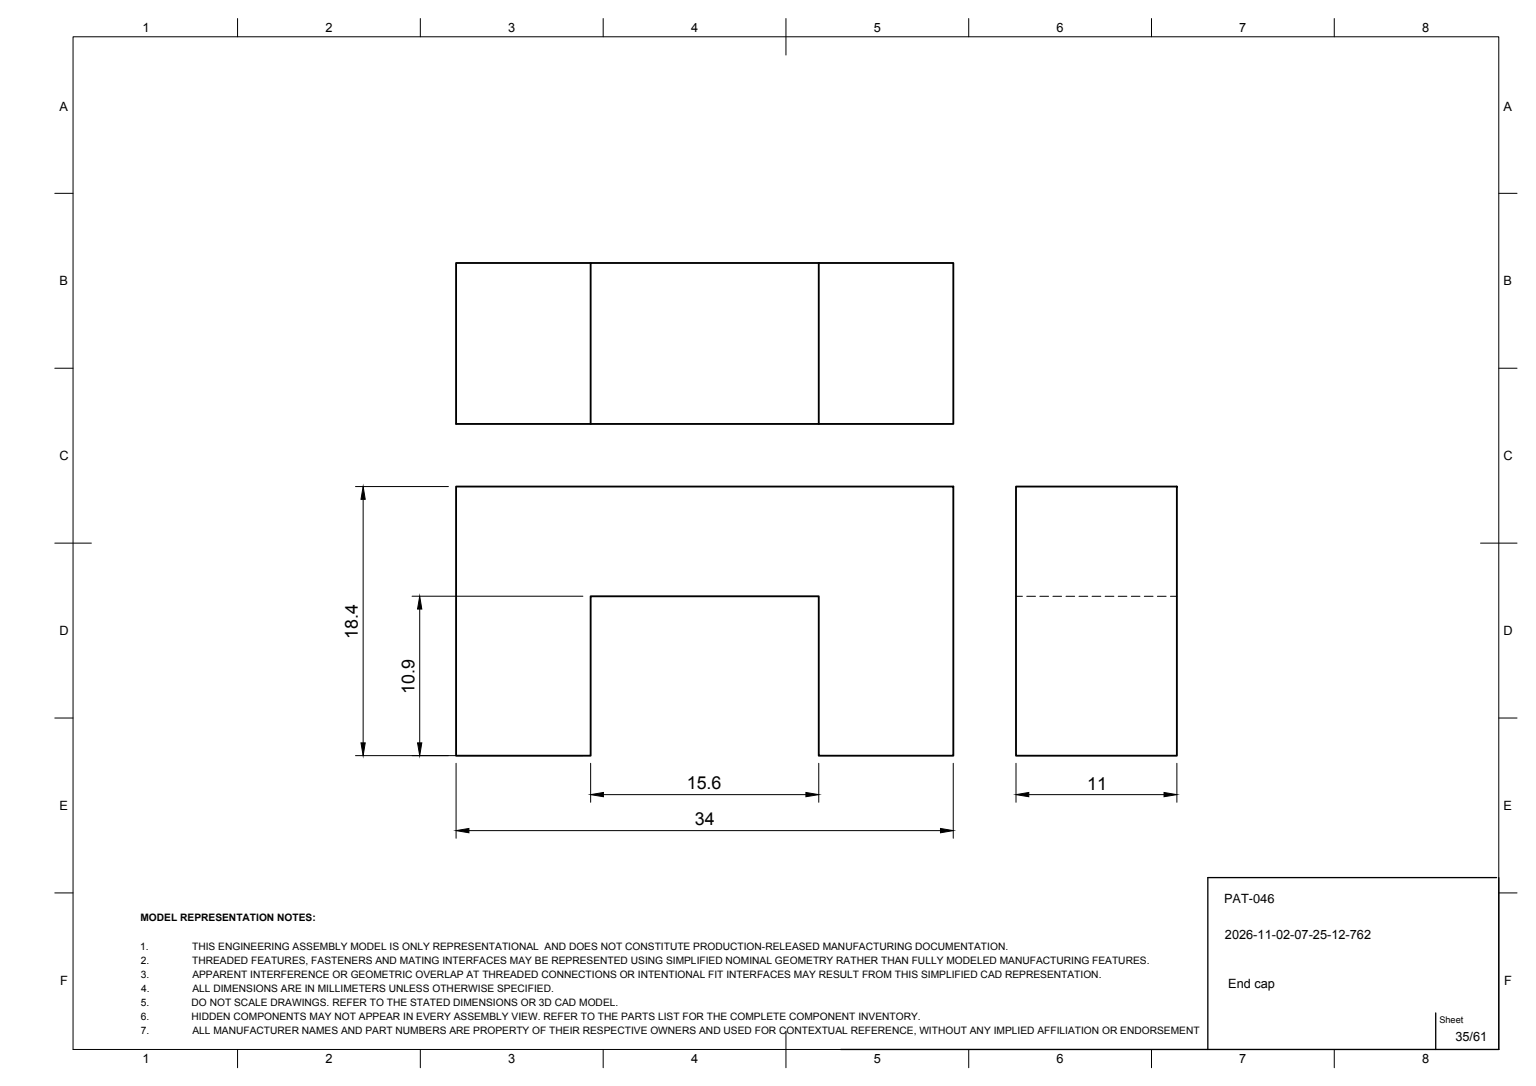
ISO-10303-21;
HEADER;
/* Generated by software containing ST-Developer
 * from STEP Tools, Inc. (www.steptools.com) 
 */

FILE_DESCRIPTION(
/* description */ ('Gear mesh backlash fixture'),
/* implementation_level */ '2;1');

FILE_NAME(
/* name */ 'End cap.step',
/* time_stamp */ '2026-10-28T03:26:00-07:00',
/* author */ (''),
/* organization */ (''),
/* preprocessor_version */ 'ST-DEVELOPER v20.2',
/* originating_system */ 'Autodesk Translation Framework v15.17.0.0',
/* authorisation */ '');

FILE_SCHEMA (('AUTOMOTIVE_DESIGN { 1 0 10303 214 3 1 1 }'));
ENDSEC;

DATA;
#10=MECHANICAL_DESIGN_GEOMETRIC_PRESENTATION_REPRESENTATION('',(#1048),#57900);
#941=SHAPE_REPRESENTATION_RELATIONSHIP('SRR','None',#58139,#991);
#991=ADVANCED_BREP_SHAPE_REPRESENTATION('',(#1112),#57872);
#1048=STYLED_ITEM('',(#58479),#1112);
#1112=MANIFOLD_SOLID_BREP('Body1',#13609);
#1502=PLANE('',#14853);
#1503=PLANE('',#14854);
#1504=PLANE('',#14855);
#1505=PLANE('',#14856);
#1506=PLANE('',#14857);
#1507=PLANE('',#14858);
#1508=PLANE('',#14859);
#1509=PLANE('',#14860);
#1510=PLANE('',#14861);
#1511=PLANE('',#14862);
#2006=FACE_OUTER_BOUND('',#2908,.T.);
#2007=FACE_OUTER_BOUND('',#2909,.T.);
#2008=FACE_OUTER_BOUND('',#2910,.T.);
#2009=FACE_OUTER_BOUND('',#2911,.T.);
#2010=FACE_OUTER_BOUND('',#2912,.T.);
#2011=FACE_OUTER_BOUND('',#2913,.T.);
#2012=FACE_OUTER_BOUND('',#2914,.T.);
#2013=FACE_OUTER_BOUND('',#2915,.T.);
#2014=FACE_OUTER_BOUND('',#2916,.T.);
#2015=FACE_OUTER_BOUND('',#2917,.T.);
#2908=EDGE_LOOP('',(#10317,#10318,#10319,#10320));
#2909=EDGE_LOOP('',(#10321,#10322,#10323,#10324));
#2910=EDGE_LOOP('',(#10325,#10326,#10327,#10328));
#2911=EDGE_LOOP('',(#10329,#10330,#10331,#10332));
#2912=EDGE_LOOP('',(#10333,#10334,#10335,#10336));
#2913=EDGE_LOOP('',(#10337,#10338,#10339,#10340));
#2914=EDGE_LOOP('',(#10341,#10342,#10343,#10344));
#2915=EDGE_LOOP('',(#10345,#10346,#10347,#10348));
#2916=EDGE_LOOP('',(#10349,#10350,#10351,#10352,#10353,#10354,#10355,#10356));
#2917=EDGE_LOOP('',(#10357,#10358,#10359,#10360,#10361,#10362,#10363,#10364));
#3795=LINE('',#21242,#4684);
#3796=LINE('',#21244,#4685);
#3797=LINE('',#21246,#4686);
#3798=LINE('',#21247,#4687);
#3799=LINE('',#21250,#4688);
#3800=LINE('',#21252,#4689);
#3801=LINE('',#21253,#4690);
#3802=LINE('',#21256,#4691);
#3803=LINE('',#21258,#4692);
#3804=LINE('',#21259,#4693);
#3805=LINE('',#21262,#4694);
#3806=LINE('',#21264,#4695);
#3807=LINE('',#21265,#4696);
#3808=LINE('',#21268,#4697);
#3809=LINE('',#21270,#4698);
#3810=LINE('',#21271,#4699);
#3811=LINE('',#21274,#4700);
#3812=LINE('',#21276,#4701);
#3813=LINE('',#21277,#4702);
#3814=LINE('',#21280,#4703);
#3815=LINE('',#21282,#4704);
#3816=LINE('',#21283,#4705);
#3817=LINE('',#21285,#4706);
#3818=LINE('',#21286,#4707);
#4684=VECTOR('',#17280,1.);
#4685=VECTOR('',#17281,1.);
#4686=VECTOR('',#17282,1.);
#4687=VECTOR('',#17283,1.);
#4688=VECTOR('',#17286,1.);
#4689=VECTOR('',#17287,1.);
#4690=VECTOR('',#17288,1.);
#4691=VECTOR('',#17291,1.);
#4692=VECTOR('',#17292,1.);
#4693=VECTOR('',#17293,1.);
#4694=VECTOR('',#17296,1.);
#4695=VECTOR('',#17297,1.);
#4696=VECTOR('',#17298,1.);
#4697=VECTOR('',#17301,1.);
#4698=VECTOR('',#17302,1.);
#4699=VECTOR('',#17303,1.);
#4700=VECTOR('',#17306,1.);
#4701=VECTOR('',#17307,1.);
#4702=VECTOR('',#17308,1.);
#4703=VECTOR('',#17311,1.);
#4704=VECTOR('',#17312,1.);
#4705=VECTOR('',#17313,1.);
#4706=VECTOR('',#17316,1.);
#4707=VECTOR('',#17317,1.);
#6263=VERTEX_POINT('',#21240);
#6264=VERTEX_POINT('',#21241);
#6265=VERTEX_POINT('',#21243);
#6266=VERTEX_POINT('',#21245);
#6267=VERTEX_POINT('',#21249);
#6268=VERTEX_POINT('',#21251);
#6269=VERTEX_POINT('',#21255);
#6270=VERTEX_POINT('',#21257);
#6271=VERTEX_POINT('',#21261);
#6272=VERTEX_POINT('',#21263);
#6273=VERTEX_POINT('',#21267);
#6274=VERTEX_POINT('',#21269);
#6275=VERTEX_POINT('',#21273);
#6276=VERTEX_POINT('',#21275);
#6277=VERTEX_POINT('',#21279);
#6278=VERTEX_POINT('',#21281);
#7745=EDGE_CURVE('',#6263,#6264,#3795,.T.);
#7746=EDGE_CURVE('',#6263,#6265,#3796,.T.);
#7747=EDGE_CURVE('',#6266,#6265,#3797,.T.);
#7748=EDGE_CURVE('',#6264,#6266,#3798,.T.);
#7749=EDGE_CURVE('',#6264,#6267,#3799,.T.);
#7750=EDGE_CURVE('',#6268,#6266,#3800,.T.);
#7751=EDGE_CURVE('',#6267,#6268,#3801,.T.);
#7752=EDGE_CURVE('',#6267,#6269,#3802,.T.);
#7753=EDGE_CURVE('',#6270,#6268,#3803,.T.);
#7754=EDGE_CURVE('',#6269,#6270,#3804,.T.);
#7755=EDGE_CURVE('',#6269,#6271,#3805,.T.);
#7756=EDGE_CURVE('',#6272,#6270,#3806,.T.);
#7757=EDGE_CURVE('',#6271,#6272,#3807,.T.);
#7758=EDGE_CURVE('',#6271,#6273,#3808,.T.);
#7759=EDGE_CURVE('',#6274,#6272,#3809,.T.);
#7760=EDGE_CURVE('',#6273,#6274,#3810,.T.);
#7761=EDGE_CURVE('',#6273,#6275,#3811,.T.);
#7762=EDGE_CURVE('',#6276,#6274,#3812,.T.);
#7763=EDGE_CURVE('',#6275,#6276,#3813,.T.);
#7764=EDGE_CURVE('',#6275,#6277,#3814,.T.);
#7765=EDGE_CURVE('',#6278,#6276,#3815,.T.);
#7766=EDGE_CURVE('',#6277,#6278,#3816,.T.);
#7767=EDGE_CURVE('',#6277,#6263,#3817,.T.);
#7768=EDGE_CURVE('',#6265,#6278,#3818,.T.);
#10317=ORIENTED_EDGE('',*,*,#7745,.F.);
#10318=ORIENTED_EDGE('',*,*,#7746,.T.);
#10319=ORIENTED_EDGE('',*,*,#7747,.F.);
#10320=ORIENTED_EDGE('',*,*,#7748,.F.);
#10321=ORIENTED_EDGE('',*,*,#7749,.F.);
#10322=ORIENTED_EDGE('',*,*,#7748,.T.);
#10323=ORIENTED_EDGE('',*,*,#7750,.F.);
#10324=ORIENTED_EDGE('',*,*,#7751,.F.);
#10325=ORIENTED_EDGE('',*,*,#7752,.F.);
#10326=ORIENTED_EDGE('',*,*,#7751,.T.);
#10327=ORIENTED_EDGE('',*,*,#7753,.F.);
#10328=ORIENTED_EDGE('',*,*,#7754,.F.);
#10329=ORIENTED_EDGE('',*,*,#7755,.F.);
#10330=ORIENTED_EDGE('',*,*,#7754,.T.);
#10331=ORIENTED_EDGE('',*,*,#7756,.F.);
#10332=ORIENTED_EDGE('',*,*,#7757,.F.);
#10333=ORIENTED_EDGE('',*,*,#7758,.F.);
#10334=ORIENTED_EDGE('',*,*,#7757,.T.);
#10335=ORIENTED_EDGE('',*,*,#7759,.F.);
#10336=ORIENTED_EDGE('',*,*,#7760,.F.);
#10337=ORIENTED_EDGE('',*,*,#7761,.F.);
#10338=ORIENTED_EDGE('',*,*,#7760,.T.);
#10339=ORIENTED_EDGE('',*,*,#7762,.F.);
#10340=ORIENTED_EDGE('',*,*,#7763,.F.);
#10341=ORIENTED_EDGE('',*,*,#7764,.F.);
#10342=ORIENTED_EDGE('',*,*,#7763,.T.);
#10343=ORIENTED_EDGE('',*,*,#7765,.F.);
#10344=ORIENTED_EDGE('',*,*,#7766,.F.);
#10345=ORIENTED_EDGE('',*,*,#7767,.F.);
#10346=ORIENTED_EDGE('',*,*,#7766,.T.);
#10347=ORIENTED_EDGE('',*,*,#7768,.F.);
#10348=ORIENTED_EDGE('',*,*,#7746,.F.);
#10349=ORIENTED_EDGE('',*,*,#7767,.T.);
#10350=ORIENTED_EDGE('',*,*,#7745,.T.);
#10351=ORIENTED_EDGE('',*,*,#7749,.T.);
#10352=ORIENTED_EDGE('',*,*,#7752,.T.);
#10353=ORIENTED_EDGE('',*,*,#7755,.T.);
#10354=ORIENTED_EDGE('',*,*,#7758,.T.);
#10355=ORIENTED_EDGE('',*,*,#7761,.T.);
#10356=ORIENTED_EDGE('',*,*,#7764,.T.);
#10357=ORIENTED_EDGE('',*,*,#7768,.T.);
#10358=ORIENTED_EDGE('',*,*,#7765,.T.);
#10359=ORIENTED_EDGE('',*,*,#7762,.T.);
#10360=ORIENTED_EDGE('',*,*,#7759,.T.);
#10361=ORIENTED_EDGE('',*,*,#7756,.T.);
#10362=ORIENTED_EDGE('',*,*,#7753,.T.);
#10363=ORIENTED_EDGE('',*,*,#7750,.T.);
#10364=ORIENTED_EDGE('',*,*,#7747,.T.);
#13123=ADVANCED_FACE('',(#2006),#1502,.T.);
#13124=ADVANCED_FACE('',(#2007),#1503,.T.);
#13125=ADVANCED_FACE('',(#2008),#1504,.T.);
#13126=ADVANCED_FACE('',(#2009),#1505,.T.);
#13127=ADVANCED_FACE('',(#2010),#1506,.T.);
#13128=ADVANCED_FACE('',(#2011),#1507,.T.);
#13129=ADVANCED_FACE('',(#2012),#1508,.T.);
#13130=ADVANCED_FACE('',(#2013),#1509,.T.);
#13131=ADVANCED_FACE('',(#2014),#1510,.T.);
#13132=ADVANCED_FACE('',(#2015),#1511,.T.);
#13609=CLOSED_SHELL('',(#13123,#13124,#13125,#13126,#13127,#13128,#13129,
#13130,#13131,#13132));
#14852=AXIS2_PLACEMENT_3D('',#21238,#17276,#17277);
#14853=AXIS2_PLACEMENT_3D('',#21239,#17278,#17279);
#14854=AXIS2_PLACEMENT_3D('',#21248,#17284,#17285);
#14855=AXIS2_PLACEMENT_3D('',#21254,#17289,#17290);
#14856=AXIS2_PLACEMENT_3D('',#21260,#17294,#17295);
#14857=AXIS2_PLACEMENT_3D('',#21266,#17299,#17300);
#14858=AXIS2_PLACEMENT_3D('',#21272,#17304,#17305);
#14859=AXIS2_PLACEMENT_3D('',#21278,#17309,#17310);
#14860=AXIS2_PLACEMENT_3D('',#21284,#17314,#17315);
#14861=AXIS2_PLACEMENT_3D('',#21287,#17318,#17319);
#14862=AXIS2_PLACEMENT_3D('',#21288,#17320,#17321);
#17276=DIRECTION('axis',(0.,0.,1.));
#17277=DIRECTION('refdir',(1.,0.,0.));
#17278=DIRECTION('center_axis',(0.,0.,-1.));
#17279=DIRECTION('ref_axis',(0.,-1.,0.));
#17280=DIRECTION('',(0.,1.,0.));
#17281=DIRECTION('',(-1.,0.,0.));
#17282=DIRECTION('',(0.,-1.,0.));
#17283=DIRECTION('',(-1.,0.,0.));
#17284=DIRECTION('center_axis',(0.,1.,0.));
#17285=DIRECTION('ref_axis',(0.,0.,-1.));
#17286=DIRECTION('',(0.,0.,1.));
#17287=DIRECTION('',(0.,0.,-1.));
#17288=DIRECTION('',(-1.,0.,0.));
#17289=DIRECTION('center_axis',(0.,0.,-1.));
#17290=DIRECTION('ref_axis',(0.,-1.,0.));
#17291=DIRECTION('',(0.,1.,0.));
#17292=DIRECTION('',(0.,-1.,0.));
#17293=DIRECTION('',(-1.,0.,0.));
#17294=DIRECTION('center_axis',(0.,-1.,0.));
#17295=DIRECTION('ref_axis',(0.,0.,1.));
#17296=DIRECTION('',(0.,0.,-1.));
#17297=DIRECTION('',(0.,0.,1.));
#17298=DIRECTION('',(-1.,0.,0.));
#17299=DIRECTION('center_axis',(0.,0.,-1.));
#17300=DIRECTION('ref_axis',(0.,-1.,0.));
#17301=DIRECTION('',(0.,1.,0.));
#17302=DIRECTION('',(0.,-1.,0.));
#17303=DIRECTION('',(-1.,0.,0.));
#17304=DIRECTION('center_axis',(0.,1.,0.));
#17305=DIRECTION('ref_axis',(0.,0.,-1.));
#17306=DIRECTION('',(0.,0.,1.));
#17307=DIRECTION('',(0.,0.,-1.));
#17308=DIRECTION('',(-1.,0.,0.));
#17309=DIRECTION('center_axis',(0.,0.,1.));
#17310=DIRECTION('ref_axis',(0.,1.,0.));
#17311=DIRECTION('',(0.,-1.,0.));
#17312=DIRECTION('',(0.,1.,0.));
#17313=DIRECTION('',(-1.,0.,0.));
#17314=DIRECTION('center_axis',(0.,-1.,0.));
#17315=DIRECTION('ref_axis',(0.,0.,1.));
#17316=DIRECTION('',(0.,0.,-1.));
#17317=DIRECTION('',(0.,0.,1.));
#17318=DIRECTION('center_axis',(1.,0.,0.));
#17319=DIRECTION('ref_axis',(0.,0.,-1.));
#17320=DIRECTION('center_axis',(-1.,0.,0.));
#17321=DIRECTION('ref_axis',(0.,0.,1.));
#21238=CARTESIAN_POINT('',(0.,0.,0.));
#21239=CARTESIAN_POINT('Origin',(-1.97,-0.78,0.46));
#21240=CARTESIAN_POINT('',(-1.97,-1.7,0.46));
#21241=CARTESIAN_POINT('',(-1.97,-0.78,0.46));
#21242=CARTESIAN_POINT('',(-1.97,-1.7,0.46));
#21243=CARTESIAN_POINT('',(-3.07,-1.7,0.46));
#21244=CARTESIAN_POINT('',(-1.97,-1.7,0.46));
#21245=CARTESIAN_POINT('',(-3.07,-0.78,0.46));
#21246=CARTESIAN_POINT('',(-3.07,-1.7,0.46));
#21247=CARTESIAN_POINT('',(-1.97,-0.78,0.46));
#21248=CARTESIAN_POINT('Origin',(-1.97,-0.78,1.55));
#21249=CARTESIAN_POINT('',(-1.97,-0.78,1.55));
#21250=CARTESIAN_POINT('',(-1.97,-0.78,0.46));
#21251=CARTESIAN_POINT('',(-3.07,-0.78,1.55));
#21252=CARTESIAN_POINT('',(-3.07,-0.78,0.46));
#21253=CARTESIAN_POINT('',(-1.97,-0.78,1.55));
#21254=CARTESIAN_POINT('Origin',(-1.97,0.78,1.55));
#21255=CARTESIAN_POINT('',(-1.97,0.78,1.55));
#21256=CARTESIAN_POINT('',(-1.97,-0.78,1.55));
#21257=CARTESIAN_POINT('',(-3.07,0.78,1.55));
#21258=CARTESIAN_POINT('',(-3.07,-0.78,1.55));
#21259=CARTESIAN_POINT('',(-1.97,0.78,1.55));
#21260=CARTESIAN_POINT('Origin',(-1.97,0.78,0.46));
#21261=CARTESIAN_POINT('',(-1.97,0.78,0.46));
#21262=CARTESIAN_POINT('',(-1.97,0.78,1.55));
#21263=CARTESIAN_POINT('',(-3.07,0.78,0.46));
#21264=CARTESIAN_POINT('',(-3.07,0.78,1.55));
#21265=CARTESIAN_POINT('',(-1.97,0.78,0.46));
#21266=CARTESIAN_POINT('Origin',(-1.97,1.7,0.46));
#21267=CARTESIAN_POINT('',(-1.97,1.7,0.46));
#21268=CARTESIAN_POINT('',(-1.97,0.78,0.46));
#21269=CARTESIAN_POINT('',(-3.07,1.7,0.46));
#21270=CARTESIAN_POINT('',(-3.07,0.78,0.46));
#21271=CARTESIAN_POINT('',(-1.97,1.7,0.46));
#21272=CARTESIAN_POINT('Origin',(-1.97,1.7,2.3));
#21273=CARTESIAN_POINT('',(-1.97,1.7,2.3));
#21274=CARTESIAN_POINT('',(-1.97,1.7,0.46));
#21275=CARTESIAN_POINT('',(-3.07,1.7,2.3));
#21276=CARTESIAN_POINT('',(-3.07,1.7,0.46));
#21277=CARTESIAN_POINT('',(-1.97,1.7,2.3));
#21278=CARTESIAN_POINT('Origin',(-1.97,-1.7,2.3));
#21279=CARTESIAN_POINT('',(-1.97,-1.7,2.3));
#21280=CARTESIAN_POINT('',(-1.97,1.7,2.3));
#21281=CARTESIAN_POINT('',(-3.07,-1.7,2.3));
#21282=CARTESIAN_POINT('',(-3.07,1.7,2.3));
#21283=CARTESIAN_POINT('',(-1.97,-1.7,2.3));
#21284=CARTESIAN_POINT('Origin',(-1.97,-1.7,0.46));
#21285=CARTESIAN_POINT('',(-1.97,-1.7,2.3));
#21286=CARTESIAN_POINT('',(-3.07,-1.7,2.3));
#21287=CARTESIAN_POINT('Origin',(-1.97,0.,1.38));
#21288=CARTESIAN_POINT('Origin',(-3.07,0.,1.38));
#57813=UNCERTAINTY_MEASURE_WITH_UNIT(LENGTH_MEASURE(0.001),#57901,
'DISTANCE_ACCURACY_VALUE',
'Maximum model space distance between geometric entities at asserted c
onnectivities');
#57841=UNCERTAINTY_MEASURE_WITH_UNIT(LENGTH_MEASURE(0.001),#57901,
'DISTANCE_ACCURACY_VALUE',
'Maximum model space distance between geometric entities at asserted c
onnectivities');
#57872=(
GEOMETRIC_REPRESENTATION_CONTEXT(3)
GLOBAL_UNCERTAINTY_ASSIGNED_CONTEXT((#57813))
GLOBAL_UNIT_ASSIGNED_CONTEXT((#57901,#57903,#57904))
REPRESENTATION_CONTEXT('','3D')
);
#57900=(
GEOMETRIC_REPRESENTATION_CONTEXT(3)
GLOBAL_UNCERTAINTY_ASSIGNED_CONTEXT((#57841))
GLOBAL_UNIT_ASSIGNED_CONTEXT((#57901,#57903,#57904))
REPRESENTATION_CONTEXT('','3D')
);
#57901=(
LENGTH_UNIT()
NAMED_UNIT(*)
SI_UNIT(.CENTI.,.METRE.)
);
#57903=(
NAMED_UNIT(*)
PLANE_ANGLE_UNIT()
SI_UNIT($,.RADIAN.)
);
#57904=(
NAMED_UNIT(*)
SI_UNIT($,.STERADIAN.)
SOLID_ANGLE_UNIT()
);
#57935=SHAPE_DEFINITION_REPRESENTATION(#57998,#58139);
#57998=PRODUCT_DEFINITION_SHAPE('',$,#58198);
#58139=SHAPE_REPRESENTATION('',(#14852),#57872);
#58167=PRODUCT_DEFINITION_CONTEXT('part definition',#58343,'design');
#58198=PRODUCT_DEFINITION('End cap','End cap',#58256,#58167);
#58256=PRODUCT_DEFINITION_FORMATION('',$,#58375);
#58343=APPLICATION_CONTEXT(
'Core Data for Automotive Mechanical Design Process');
#58344=PRODUCT_CONTEXT('part definition',#58343,'mechanical');
#58375=PRODUCT('End cap','End cap','End cap',(#58344));
#58473=COLOUR_RGB('Off White',0.89,0.88,0.83);
#58474=FILL_AREA_STYLE_COLOUR('',#58473);
#58475=FILL_AREA_STYLE('',(#58474));
#58476=SURFACE_STYLE_FILL_AREA(#58475);
#58477=SURFACE_SIDE_STYLE('',(#58476));
#58478=SURFACE_STYLE_USAGE(.BOTH.,#58477);
#58479=PRESENTATION_STYLE_ASSIGNMENT((#58478));
ENDSEC;
END-ISO-10303-21;
